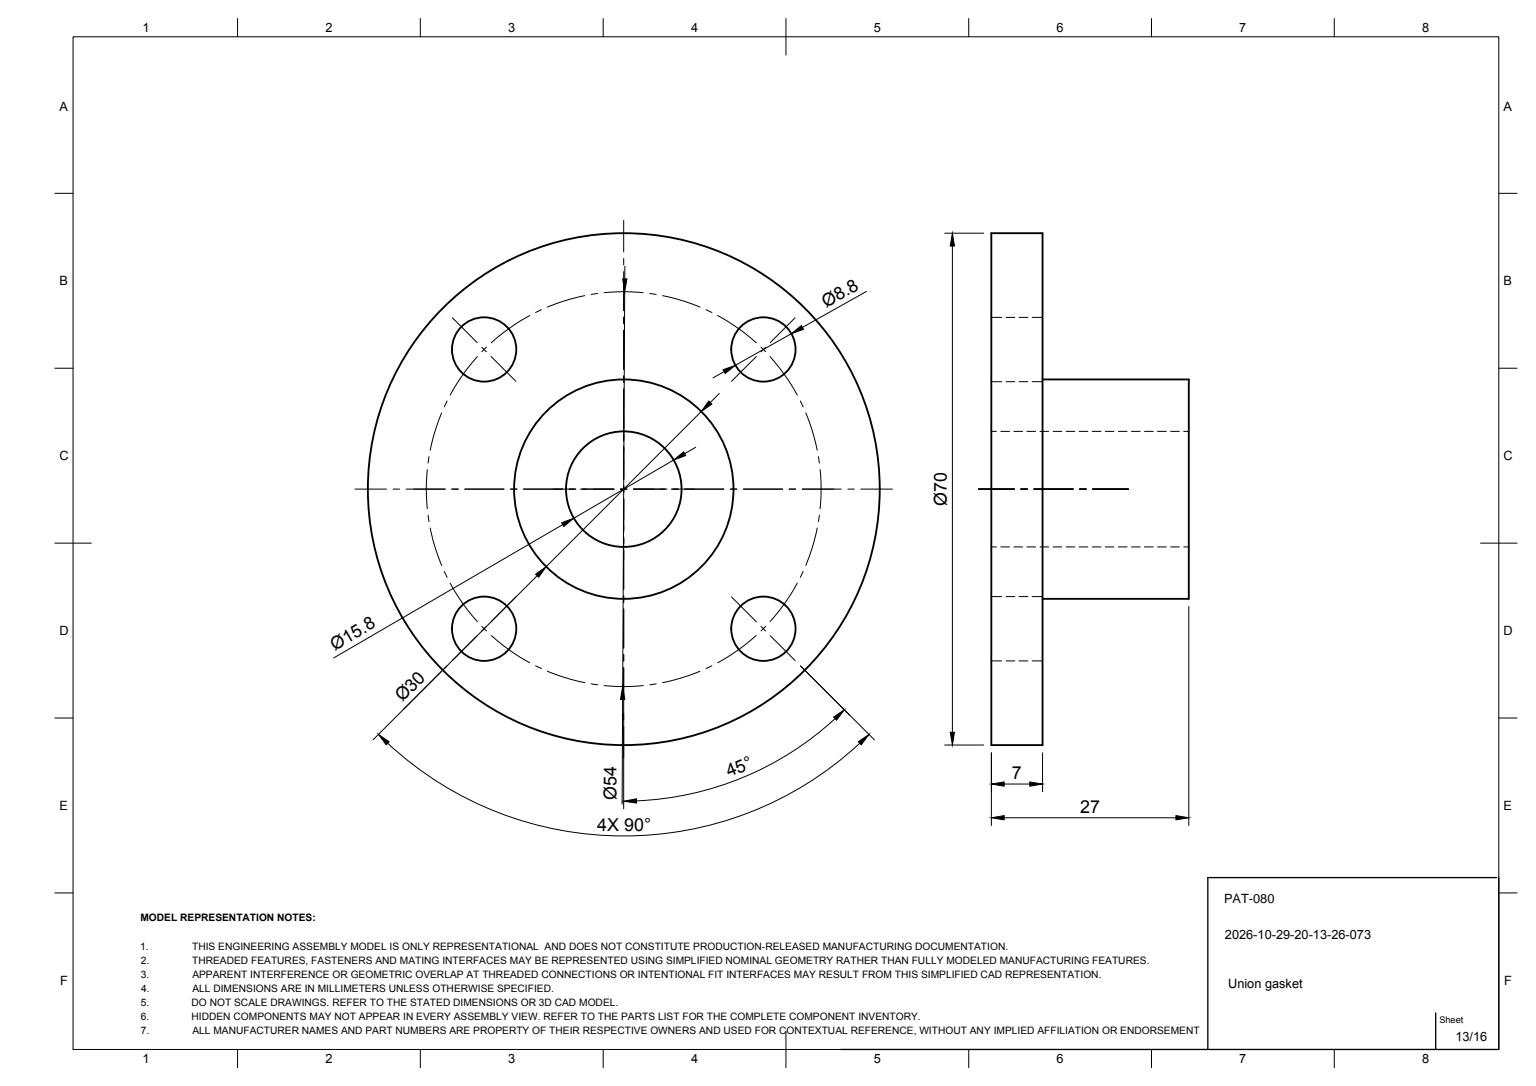
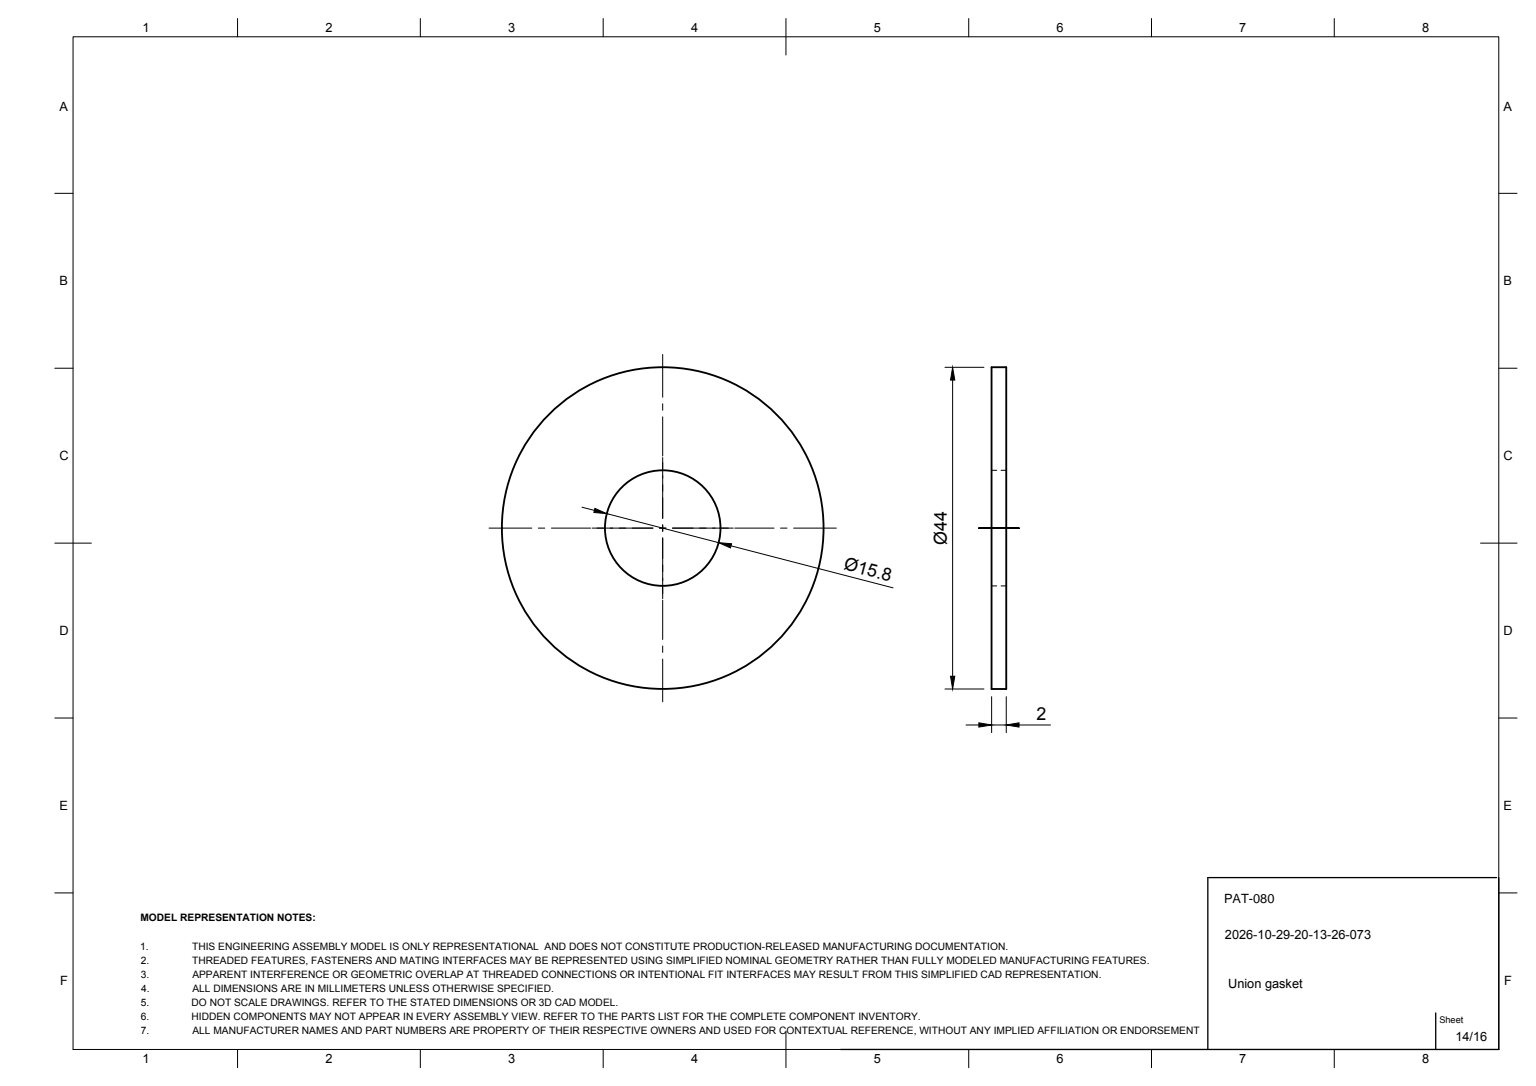
ISO-10303-21;
HEADER;
/* Generated by software containing ST-Developer
 * from STEP Tools, Inc. (www.steptools.com) 
 */

FILE_DESCRIPTION(
/* description */ ('PAT-080'),
/* implementation_level */ '2;1');

FILE_NAME(
/* name */ 'Union gasket.step',
/* time_stamp */ '2026-10-29T20:13:47-07:00',
/* author */ (''),
/* organization */ (''),
/* preprocessor_version */ 'ST-DEVELOPER v20.2',
/* originating_system */ 'Autodesk Translation Framework v15.17.0.0',
/* authorisation */ '');

FILE_SCHEMA (('AUTOMOTIVE_DESIGN { 1 0 10303 214 3 1 1 }'));
ENDSEC;

DATA;
#10=MECHANICAL_DESIGN_GEOMETRIC_PRESENTATION_REPRESENTATION('',(#257),#6878);
#219=SHAPE_REPRESENTATION_RELATIONSHIP('SRR','None',#6975,#238);
#238=ADVANCED_BREP_SHAPE_REPRESENTATION('',(#276),#6870);
#257=STYLED_ITEM('',(#7115),#276);
#276=MANIFOLD_SOLID_BREP('Body1',#3873);
#337=FACE_BOUND('',#911,.T.);
#338=FACE_BOUND('',#913,.T.);
#439=PLANE('',#4327);
#440=PLANE('',#4328);
#626=FACE_OUTER_BOUND('',#908,.T.);
#627=FACE_OUTER_BOUND('',#909,.T.);
#628=FACE_OUTER_BOUND('',#910,.T.);
#629=FACE_OUTER_BOUND('',#912,.T.);
#908=EDGE_LOOP('',(#3184,#3185,#3186,#3187));
#909=EDGE_LOOP('',(#3188,#3189,#3190,#3191));
#910=EDGE_LOOP('',(#3192));
#911=EDGE_LOOP('',(#3193));
#912=EDGE_LOOP('',(#3194));
#913=EDGE_LOOP('',(#3195));
#1228=LINE('',#6352,#1543);
#1229=LINE('',#6358,#1544);
#1543=VECTOR('',#5192,0.79);
#1544=VECTOR('',#5199,2.2);
#1746=CIRCLE('',#4322,0.79);
#1747=CIRCLE('',#4323,0.79);
#1748=CIRCLE('',#4325,2.2);
#1749=CIRCLE('',#4326,2.2);
#2002=VERTEX_POINT('',#6349);
#2003=VERTEX_POINT('',#6351);
#2004=VERTEX_POINT('',#6355);
#2005=VERTEX_POINT('',#6357);
#2415=EDGE_CURVE('',#2002,#2002,#1746,.T.);
#2416=EDGE_CURVE('',#2002,#2003,#1228,.T.);
#2417=EDGE_CURVE('',#2003,#2003,#1747,.T.);
#2418=EDGE_CURVE('',#2004,#2004,#1748,.T.);
#2419=EDGE_CURVE('',#2004,#2005,#1229,.T.);
#2420=EDGE_CURVE('',#2005,#2005,#1749,.T.);
#3184=ORIENTED_EDGE('',*,*,#2415,.F.);
#3185=ORIENTED_EDGE('',*,*,#2416,.T.);
#3186=ORIENTED_EDGE('',*,*,#2417,.T.);
#3187=ORIENTED_EDGE('',*,*,#2416,.F.);
#3188=ORIENTED_EDGE('',*,*,#2418,.F.);
#3189=ORIENTED_EDGE('',*,*,#2419,.T.);
#3190=ORIENTED_EDGE('',*,*,#2420,.T.);
#3191=ORIENTED_EDGE('',*,*,#2419,.F.);
#3192=ORIENTED_EDGE('',*,*,#2418,.T.);
#3193=ORIENTED_EDGE('',*,*,#2415,.T.);
#3194=ORIENTED_EDGE('',*,*,#2420,.F.);
#3195=ORIENTED_EDGE('',*,*,#2417,.F.);
#3614=CYLINDRICAL_SURFACE('',#4321,0.79);
#3615=CYLINDRICAL_SURFACE('',#4324,2.2);
#3762=ADVANCED_FACE('',(#626),#3614,.F.);
#3763=ADVANCED_FACE('',(#627),#3615,.T.);
#3764=ADVANCED_FACE('',(#628,#337),#439,.T.);
#3765=ADVANCED_FACE('',(#629,#338),#440,.F.);
#3873=CLOSED_SHELL('',(#3762,#3763,#3764,#3765));
#4320=AXIS2_PLACEMENT_3D('',#6347,#5186,#5187);
#4321=AXIS2_PLACEMENT_3D('',#6348,#5188,#5189);
#4322=AXIS2_PLACEMENT_3D('',#6350,#5190,#5191);
#4323=AXIS2_PLACEMENT_3D('',#6353,#5193,#5194);
#4324=AXIS2_PLACEMENT_3D('',#6354,#5195,#5196);
#4325=AXIS2_PLACEMENT_3D('',#6356,#5197,#5198);
#4326=AXIS2_PLACEMENT_3D('',#6359,#5200,#5201);
#4327=AXIS2_PLACEMENT_3D('',#6360,#5202,#5203);
#4328=AXIS2_PLACEMENT_3D('',#6361,#5204,#5205);
#5186=DIRECTION('axis',(0.,0.,1.));
#5187=DIRECTION('refdir',(1.,0.,0.));
#5188=DIRECTION('center_axis',(1.,0.,0.));
#5189=DIRECTION('ref_axis',(0.,0.,-1.));
#5190=DIRECTION('center_axis',(-1.,0.,0.));
#5191=DIRECTION('ref_axis',(0.,0.,-1.));
#5192=DIRECTION('',(-1.,0.,0.));
#5193=DIRECTION('center_axis',(-1.,0.,0.));
#5194=DIRECTION('ref_axis',(0.,0.,-1.));
#5195=DIRECTION('center_axis',(1.,0.,0.));
#5196=DIRECTION('ref_axis',(0.,0.,-1.));
#5197=DIRECTION('center_axis',(1.,0.,0.));
#5198=DIRECTION('ref_axis',(0.,0.,-1.));
#5199=DIRECTION('',(-1.,0.,0.));
#5200=DIRECTION('center_axis',(1.,0.,0.));
#5201=DIRECTION('ref_axis',(0.,0.,-1.));
#5202=DIRECTION('center_axis',(1.,0.,0.));
#5203=DIRECTION('ref_axis',(0.,0.,-1.));
#5204=DIRECTION('center_axis',(1.,0.,0.));
#5205=DIRECTION('ref_axis',(0.,0.,-1.));
#6347=CARTESIAN_POINT('',(0.,0.,0.));
#6348=CARTESIAN_POINT('Origin',(-0.1,0.,6.));
#6349=CARTESIAN_POINT('',(0.1,-9.67470971326409E-17,6.79));
#6350=CARTESIAN_POINT('Origin',(0.1,0.,6.));
#6351=CARTESIAN_POINT('',(-0.1,-9.67470971326409E-17,6.79));
#6352=CARTESIAN_POINT('',(-0.1,-9.67470971326409E-17,6.79));
#6353=CARTESIAN_POINT('Origin',(-0.1,0.,6.));
#6354=CARTESIAN_POINT('Origin',(-0.1,0.,6.));
#6355=CARTESIAN_POINT('',(0.1,-2.69422295812418E-16,8.2));
#6356=CARTESIAN_POINT('Origin',(0.1,0.,6.));
#6357=CARTESIAN_POINT('',(-0.1,-2.69422295812418E-16,8.2));
#6358=CARTESIAN_POINT('',(-0.1,-2.69422295812418E-16,8.2));
#6359=CARTESIAN_POINT('Origin',(-0.1,0.,6.));
#6360=CARTESIAN_POINT('Origin',(0.1,0.,6.));
#6361=CARTESIAN_POINT('Origin',(-0.1,0.,6.));
#6849=UNCERTAINTY_MEASURE_WITH_UNIT(LENGTH_MEASURE(0.001),#6879,
'DISTANCE_ACCURACY_VALUE',
'Maximum model space distance between geometric entities at asserted c
onnectivities');
#6857=UNCERTAINTY_MEASURE_WITH_UNIT(LENGTH_MEASURE(0.001),#6879,
'DISTANCE_ACCURACY_VALUE',
'Maximum model space distance between geometric entities at asserted c
onnectivities');
#6870=(
GEOMETRIC_REPRESENTATION_CONTEXT(3)
GLOBAL_UNCERTAINTY_ASSIGNED_CONTEXT((#6849))
GLOBAL_UNIT_ASSIGNED_CONTEXT((#6879,#6881,#6882))
REPRESENTATION_CONTEXT('','3D')
);
#6878=(
GEOMETRIC_REPRESENTATION_CONTEXT(3)
GLOBAL_UNCERTAINTY_ASSIGNED_CONTEXT((#6857))
GLOBAL_UNIT_ASSIGNED_CONTEXT((#6879,#6881,#6882))
REPRESENTATION_CONTEXT('','3D')
);
#6879=(
LENGTH_UNIT()
NAMED_UNIT(*)
SI_UNIT(.CENTI.,.METRE.)
);
#6881=(
NAMED_UNIT(*)
PLANE_ANGLE_UNIT()
SI_UNIT($,.RADIAN.)
);
#6882=(
NAMED_UNIT(*)
SI_UNIT($,.STERADIAN.)
SOLID_ANGLE_UNIT()
);
#6895=SHAPE_DEFINITION_REPRESENTATION(#6915,#6975);
#6915=PRODUCT_DEFINITION_SHAPE('',$,#6996);
#6975=SHAPE_REPRESENTATION('',(#4320),#6870);
#6983=PRODUCT_DEFINITION_CONTEXT('part definition',#7045,'design');
#6996=PRODUCT_DEFINITION('Union gasket','Union gasket',#7016,
#6983);
#7016=PRODUCT_DEFINITION_FORMATION('',$,#7059);
#7045=APPLICATION_CONTEXT(
'Core Data for Automotive Mechanical Design Process');
#7046=PRODUCT_CONTEXT('part definition',#7045,'mechanical');
#7059=PRODUCT('Union gasket','Union gasket','Union gasket',(#7046));
#7109=COLOUR_RGB('Light Blue',0.38,0.62,0.78);
#7110=FILL_AREA_STYLE_COLOUR('',#7109);
#7111=FILL_AREA_STYLE('',(#7110));
#7112=SURFACE_STYLE_FILL_AREA(#7111);
#7113=SURFACE_SIDE_STYLE('',(#7112));
#7114=SURFACE_STYLE_USAGE(.BOTH.,#7113);
#7115=PRESENTATION_STYLE_ASSIGNMENT((#7114));
ENDSEC;
END-ISO-10303-21;
